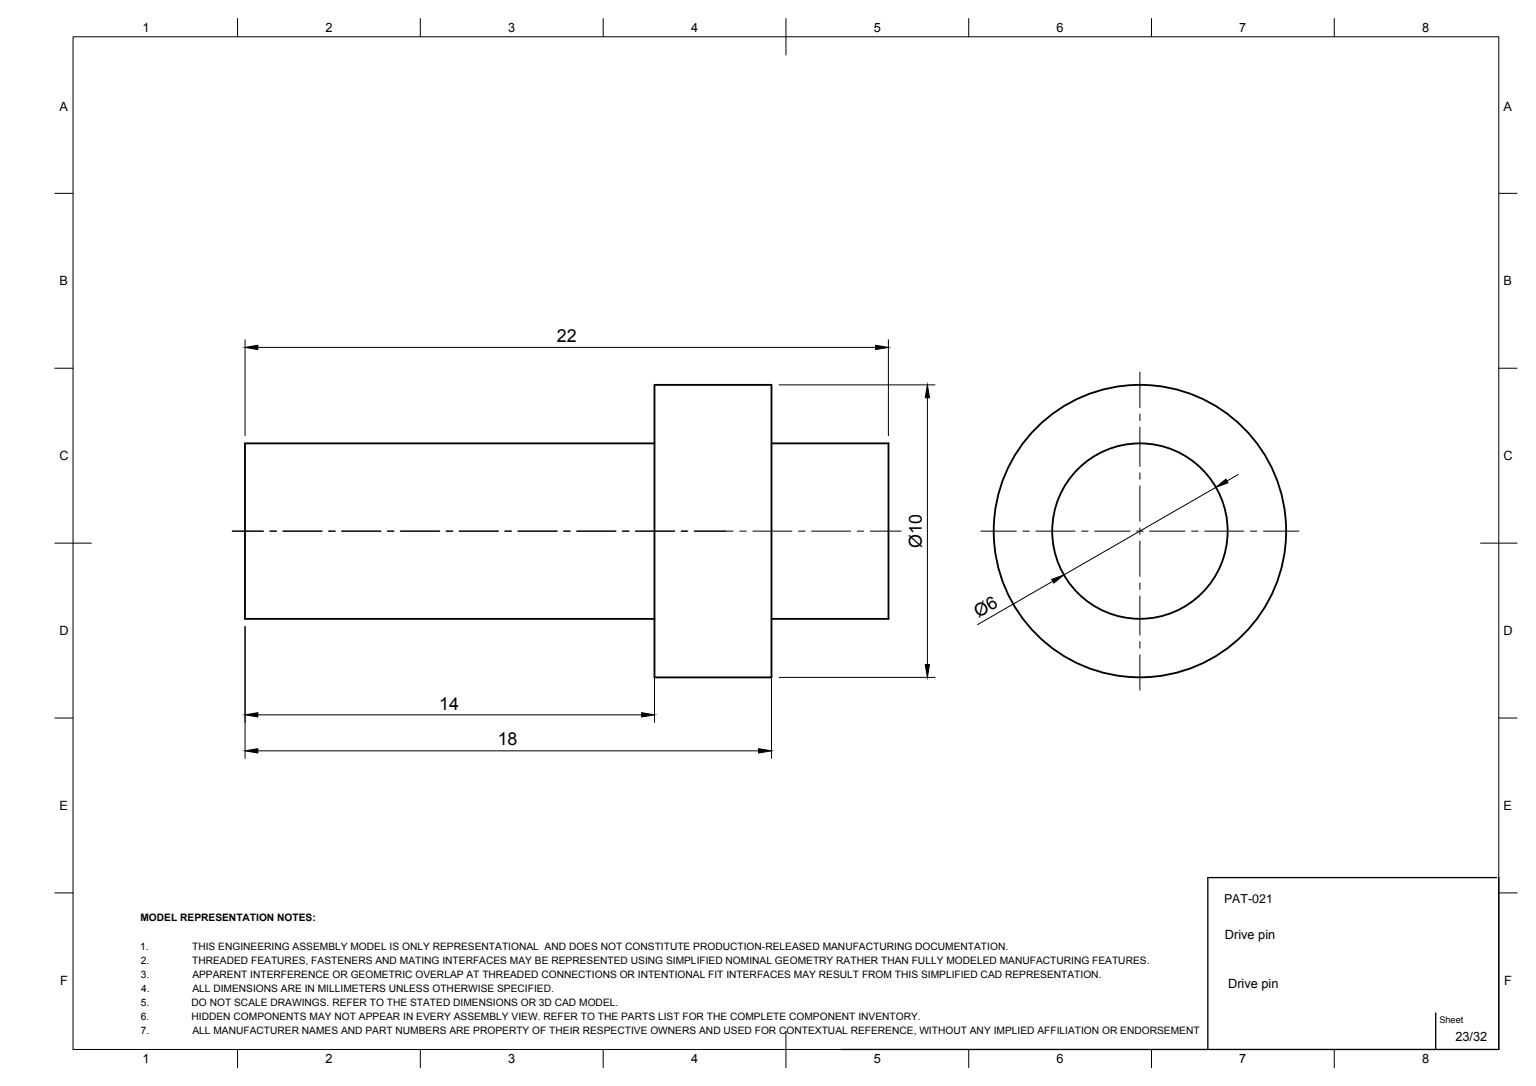
ISO-10303-21;
HEADER;
/* Generated by software containing ST-Developer
 * from STEP Tools, Inc. (www.steptools.com) 
 */

FILE_DESCRIPTION(
/* description */ ('Chain-less indexing wheel (Geneva) drive'),
/* implementation_level */ '2;1');

FILE_NAME(
/* name */ 'Drive pin.step',
/* time_stamp */ '2026-10-28T03:25:22-07:00',
/* author */ (''),
/* organization */ (''),
/* preprocessor_version */ 'ST-DEVELOPER v20.2',
/* originating_system */ 'Autodesk Translation Framework v15.17.0.0',
/* authorisation */ '');

FILE_SCHEMA (('AUTOMOTIVE_DESIGN { 1 0 10303 214 3 1 1 }'));
ENDSEC;

DATA;
#10=MECHANICAL_DESIGN_GEOMETRIC_PRESENTATION_REPRESENTATION('',(#326),#10957);
#268=SHAPE_REPRESENTATION_RELATIONSHIP('SRR','None',#11083,#293);
#293=ADVANCED_BREP_SHAPE_REPRESENTATION('',(#358),#10946);
#326=STYLED_ITEM('',(#11287),#358);
#358=MANIFOLD_SOLID_BREP('Body1',#5723);
#445=FACE_BOUND('',#1273,.T.);
#446=FACE_BOUND('',#1275,.T.);
#575=PLANE('',#6471);
#576=PLANE('',#6474);
#577=PLANE('',#6482);
#578=PLANE('',#6483);
#861=FACE_OUTER_BOUND('',#1272,.T.);
#862=FACE_OUTER_BOUND('',#1274,.T.);
#863=FACE_OUTER_BOUND('',#1276,.T.);
#864=FACE_OUTER_BOUND('',#1277,.T.);
#865=FACE_OUTER_BOUND('',#1278,.T.);
#866=FACE_OUTER_BOUND('',#1279,.T.);
#867=FACE_OUTER_BOUND('',#1280,.T.);
#1272=EDGE_LOOP('',(#4659));
#1273=EDGE_LOOP('',(#4660));
#1274=EDGE_LOOP('',(#4661));
#1275=EDGE_LOOP('',(#4662));
#1276=EDGE_LOOP('',(#4663,#4664,#4665,#4666));
#1277=EDGE_LOOP('',(#4667,#4668,#4669,#4670));
#1278=EDGE_LOOP('',(#4671,#4672,#4673,#4674));
#1279=EDGE_LOOP('',(#4675));
#1280=EDGE_LOOP('',(#4676));
#1622=LINE('',#10129,#1996);
#1623=LINE('',#10132,#1997);
#1624=LINE('',#10137,#1998);
#1996=VECTOR('',#7884,0.5);
#1997=VECTOR('',#7887,0.3);
#1998=VECTOR('',#7894,0.3);
#2398=CIRCLE('',#6472,0.5);
#2399=CIRCLE('',#6473,0.3);
#2400=CIRCLE('',#6475,0.5);
#2401=CIRCLE('',#6476,0.3);
#2402=CIRCLE('',#6479,0.3);
#2403=CIRCLE('',#6481,0.3);
#2806=VERTEX_POINT('',#10119);
#2807=VERTEX_POINT('',#10121);
#2808=VERTEX_POINT('',#10124);
#2809=VERTEX_POINT('',#10126);
#2810=VERTEX_POINT('',#10131);
#2811=VERTEX_POINT('',#10135);
#3455=EDGE_CURVE('',#2806,#2806,#2398,.T.);
#3456=EDGE_CURVE('',#2807,#2807,#2399,.T.);
#3457=EDGE_CURVE('',#2808,#2808,#2400,.T.);
#3458=EDGE_CURVE('',#2809,#2809,#2401,.T.);
#3459=EDGE_CURVE('',#2806,#2808,#1622,.T.);
#3460=EDGE_CURVE('',#2809,#2810,#1623,.T.);
#3461=EDGE_CURVE('',#2810,#2810,#2402,.T.);
#3462=EDGE_CURVE('',#2811,#2811,#2403,.T.);
#3463=EDGE_CURVE('',#2811,#2807,#1624,.T.);
#4659=ORIENTED_EDGE('',*,*,#3455,.T.);
#4660=ORIENTED_EDGE('',*,*,#3456,.F.);
#4661=ORIENTED_EDGE('',*,*,#3457,.F.);
#4662=ORIENTED_EDGE('',*,*,#3458,.F.);
#4663=ORIENTED_EDGE('',*,*,#3455,.F.);
#4664=ORIENTED_EDGE('',*,*,#3459,.T.);
#4665=ORIENTED_EDGE('',*,*,#3457,.T.);
#4666=ORIENTED_EDGE('',*,*,#3459,.F.);
#4667=ORIENTED_EDGE('',*,*,#3458,.T.);
#4668=ORIENTED_EDGE('',*,*,#3460,.T.);
#4669=ORIENTED_EDGE('',*,*,#3461,.T.);
#4670=ORIENTED_EDGE('',*,*,#3460,.F.);
#4671=ORIENTED_EDGE('',*,*,#3462,.F.);
#4672=ORIENTED_EDGE('',*,*,#3463,.T.);
#4673=ORIENTED_EDGE('',*,*,#3456,.T.);
#4674=ORIENTED_EDGE('',*,*,#3463,.F.);
#4675=ORIENTED_EDGE('',*,*,#3462,.T.);
#4676=ORIENTED_EDGE('',*,*,#3461,.F.);
#5323=CYLINDRICAL_SURFACE('',#6477,0.5);
#5324=CYLINDRICAL_SURFACE('',#6478,0.3);
#5325=CYLINDRICAL_SURFACE('',#6480,0.3);
#5575=ADVANCED_FACE('',(#861,#445),#575,.T.);
#5576=ADVANCED_FACE('',(#862,#446),#576,.F.);
#5577=ADVANCED_FACE('',(#863),#5323,.T.);
#5578=ADVANCED_FACE('',(#864),#5324,.T.);
#5579=ADVANCED_FACE('',(#865),#5325,.T.);
#5580=ADVANCED_FACE('',(#866),#577,.T.);
#5581=ADVANCED_FACE('',(#867),#578,.F.);
#5723=CLOSED_SHELL('',(#5575,#5576,#5577,#5578,#5579,#5580,#5581));
#6470=AXIS2_PLACEMENT_3D('',#10117,#7868,#7869);
#6471=AXIS2_PLACEMENT_3D('',#10118,#7870,#7871);
#6472=AXIS2_PLACEMENT_3D('',#10120,#7872,#7873);
#6473=AXIS2_PLACEMENT_3D('',#10122,#7874,#7875);
#6474=AXIS2_PLACEMENT_3D('',#10123,#7876,#7877);
#6475=AXIS2_PLACEMENT_3D('',#10125,#7878,#7879);
#6476=AXIS2_PLACEMENT_3D('',#10127,#7880,#7881);
#6477=AXIS2_PLACEMENT_3D('',#10128,#7882,#7883);
#6478=AXIS2_PLACEMENT_3D('',#10130,#7885,#7886);
#6479=AXIS2_PLACEMENT_3D('',#10133,#7888,#7889);
#6480=AXIS2_PLACEMENT_3D('',#10134,#7890,#7891);
#6481=AXIS2_PLACEMENT_3D('',#10136,#7892,#7893);
#6482=AXIS2_PLACEMENT_3D('',#10138,#7895,#7896);
#6483=AXIS2_PLACEMENT_3D('',#10139,#7897,#7898);
#7868=DIRECTION('axis',(0.,0.,1.));
#7869=DIRECTION('refdir',(1.,0.,0.));
#7870=DIRECTION('center_axis',(0.,0.,1.));
#7871=DIRECTION('ref_axis',(1.,0.,0.));
#7872=DIRECTION('center_axis',(0.,0.,1.));
#7873=DIRECTION('ref_axis',(1.,0.,0.));
#7874=DIRECTION('center_axis',(0.,0.,1.));
#7875=DIRECTION('ref_axis',(1.,0.,0.));
#7876=DIRECTION('center_axis',(0.,0.,1.));
#7877=DIRECTION('ref_axis',(1.,0.,0.));
#7878=DIRECTION('center_axis',(0.,0.,1.));
#7879=DIRECTION('ref_axis',(1.,0.,0.));
#7880=DIRECTION('center_axis',(0.,0.,-1.));
#7881=DIRECTION('ref_axis',(1.,0.,0.));
#7882=DIRECTION('center_axis',(0.,0.,1.));
#7883=DIRECTION('ref_axis',(1.,0.,0.));
#7884=DIRECTION('',(0.,0.,-1.));
#7885=DIRECTION('center_axis',(0.,0.,1.));
#7886=DIRECTION('ref_axis',(1.,0.,0.));
#7887=DIRECTION('',(0.,0.,-1.));
#7888=DIRECTION('center_axis',(0.,0.,1.));
#7889=DIRECTION('ref_axis',(1.,0.,0.));
#7890=DIRECTION('center_axis',(0.,0.,1.));
#7891=DIRECTION('ref_axis',(1.,0.,0.));
#7892=DIRECTION('center_axis',(0.,0.,1.));
#7893=DIRECTION('ref_axis',(1.,0.,0.));
#7894=DIRECTION('',(0.,0.,-1.));
#7895=DIRECTION('center_axis',(0.,0.,1.));
#7896=DIRECTION('ref_axis',(1.,0.,0.));
#7897=DIRECTION('center_axis',(0.,0.,1.));
#7898=DIRECTION('ref_axis',(1.,0.,0.));
#10117=CARTESIAN_POINT('',(0.,0.,0.));
#10118=CARTESIAN_POINT('Origin',(3.,0.,5.6));
#10119=CARTESIAN_POINT('',(2.5,-6.12323399573677E-17,5.6));
#10120=CARTESIAN_POINT('Origin',(3.,0.,5.6));
#10121=CARTESIAN_POINT('',(2.7,-3.67394039744206E-17,5.6));
#10122=CARTESIAN_POINT('Origin',(3.,0.,5.6));
#10123=CARTESIAN_POINT('Origin',(3.,0.,5.2));
#10124=CARTESIAN_POINT('',(2.5,-6.12323399573677E-17,5.2));
#10125=CARTESIAN_POINT('Origin',(3.,0.,5.2));
#10126=CARTESIAN_POINT('',(2.7,3.67394039744206E-17,5.2));
#10127=CARTESIAN_POINT('Origin',(3.,0.,5.2));
#10128=CARTESIAN_POINT('Origin',(3.,0.,5.2));
#10129=CARTESIAN_POINT('',(2.5,-6.12323399573677E-17,5.2));
#10130=CARTESIAN_POINT('Origin',(3.,0.,4.8));
#10131=CARTESIAN_POINT('',(2.7,-3.67394039744206E-17,4.8));
#10132=CARTESIAN_POINT('',(2.7,-3.67394039744206E-17,4.8));
#10133=CARTESIAN_POINT('Origin',(3.,0.,4.8));
#10134=CARTESIAN_POINT('Origin',(3.,0.,4.8));
#10135=CARTESIAN_POINT('',(2.7,-3.67394039744206E-17,7.));
#10136=CARTESIAN_POINT('Origin',(3.,0.,7.));
#10137=CARTESIAN_POINT('',(2.7,-3.67394039744206E-17,4.8));
#10138=CARTESIAN_POINT('Origin',(3.,0.,7.));
#10139=CARTESIAN_POINT('Origin',(3.,0.,4.8));
#10915=UNCERTAINTY_MEASURE_WITH_UNIT(LENGTH_MEASURE(0.001),#10958,
'DISTANCE_ACCURACY_VALUE',
'Maximum model space distance between geometric entities at asserted c
onnectivities');
#10926=UNCERTAINTY_MEASURE_WITH_UNIT(LENGTH_MEASURE(0.001),#10958,
'DISTANCE_ACCURACY_VALUE',
'Maximum model space distance between geometric entities at asserted c
onnectivities');
#10946=(
GEOMETRIC_REPRESENTATION_CONTEXT(3)
GLOBAL_UNCERTAINTY_ASSIGNED_CONTEXT((#10915))
GLOBAL_UNIT_ASSIGNED_CONTEXT((#10958,#10960,#10961))
REPRESENTATION_CONTEXT('','3D')
);
#10957=(
GEOMETRIC_REPRESENTATION_CONTEXT(3)
GLOBAL_UNCERTAINTY_ASSIGNED_CONTEXT((#10926))
GLOBAL_UNIT_ASSIGNED_CONTEXT((#10958,#10960,#10961))
REPRESENTATION_CONTEXT('','3D')
);
#10958=(
LENGTH_UNIT()
NAMED_UNIT(*)
SI_UNIT(.CENTI.,.METRE.)
);
#10960=(
NAMED_UNIT(*)
PLANE_ANGLE_UNIT()
SI_UNIT($,.RADIAN.)
);
#10961=(
NAMED_UNIT(*)
SI_UNIT($,.STERADIAN.)
SOLID_ANGLE_UNIT()
);
#10981=SHAPE_DEFINITION_REPRESENTATION(#11016,#11083);
#11016=PRODUCT_DEFINITION_SHAPE('',$,#11114);
#11083=SHAPE_REPRESENTATION('',(#6470),#10946);
#11094=PRODUCT_DEFINITION_CONTEXT('part definition',#11186,'design');
#11114=PRODUCT_DEFINITION('Drive pin','Drive pin',#11144,#11094);
#11144=PRODUCT_DEFINITION_FORMATION('',$,#11207);
#11186=APPLICATION_CONTEXT(
'Core Data for Automotive Mechanical Design Process');
#11187=PRODUCT_CONTEXT('part definition',#11186,'mechanical');
#11207=PRODUCT('Drive pin','Drive pin','Drive pin',(#11187));
#11281=COLOUR_RGB('Grey',0.48,0.52,0.57);
#11282=FILL_AREA_STYLE_COLOUR('',#11281);
#11283=FILL_AREA_STYLE('',(#11282));
#11284=SURFACE_STYLE_FILL_AREA(#11283);
#11285=SURFACE_SIDE_STYLE('',(#11284));
#11286=SURFACE_STYLE_USAGE(.BOTH.,#11285);
#11287=PRESENTATION_STYLE_ASSIGNMENT((#11286));
ENDSEC;
END-ISO-10303-21;
